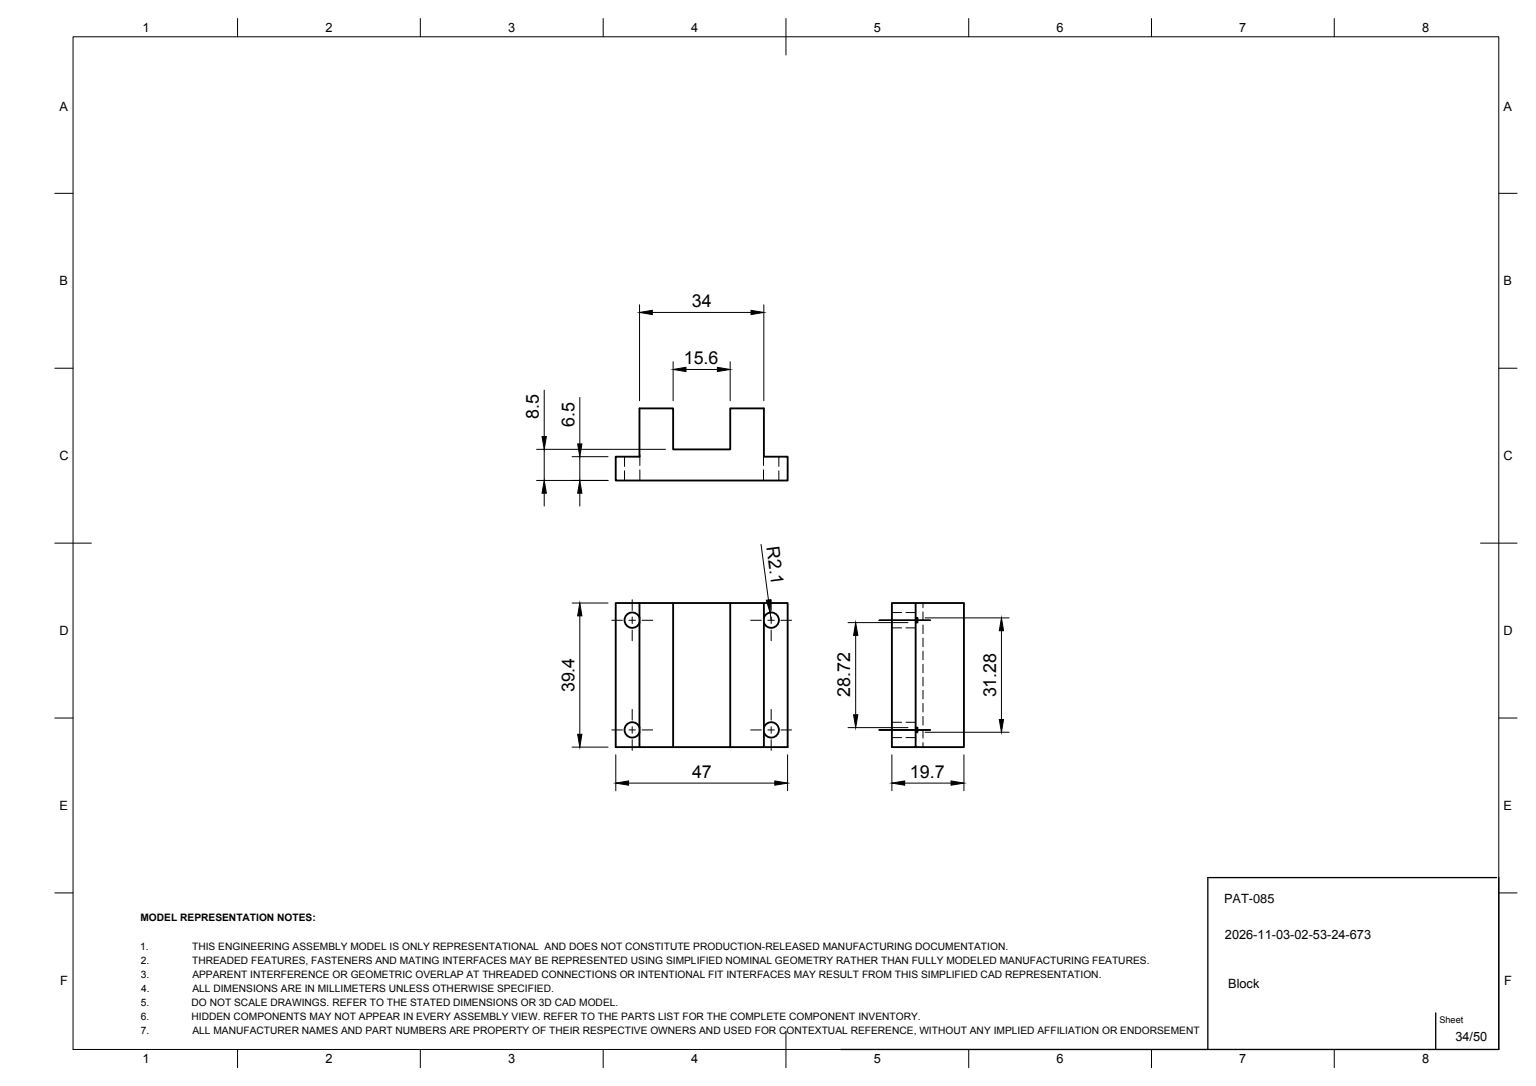
ISO-10303-21;
HEADER;
/* Generated by software containing ST-Developer
 * from STEP Tools, Inc. (www.steptools.com) 
 */

FILE_DESCRIPTION(
/* description */ ('Rack and pinion manual slide'),
/* implementation_level */ '2;1');

FILE_NAME(
/* name */ 'Block.step',
/* time_stamp */ '2026-10-28T03:22:49-07:00',
/* author */ (''),
/* organization */ (''),
/* preprocessor_version */ 'ST-DEVELOPER v20.2',
/* originating_system */ 'Autodesk Translation Framework v15.17.0.0',
/* authorisation */ '');

FILE_SCHEMA (('AUTOMOTIVE_DESIGN { 1 0 10303 214 3 1 1 }'));
ENDSEC;

DATA;
#10=MECHANICAL_DESIGN_GEOMETRIC_PRESENTATION_REPRESENTATION('',(#766),#34851);
#667=SHAPE_REPRESENTATION_RELATIONSHIP('SRR','None',#35105,#713);
#713=ADVANCED_BREP_SHAPE_REPRESENTATION('',(#817),#34830);
#766=STYLED_ITEM('',(#35390),#817);
#817=MANIFOLD_SOLID_BREP('Body1',#13788);
#1005=FACE_BOUND('',#2939,.T.);
#1006=FACE_BOUND('',#2940,.T.);
#1007=FACE_BOUND('',#2941,.T.);
#1008=FACE_BOUND('',#2942,.T.);
#1385=PLANE('',#15111);
#1386=PLANE('',#15117);
#1387=PLANE('',#15123);
#1388=PLANE('',#15129);
#1389=PLANE('',#15135);
#1390=PLANE('',#15136);
#1391=PLANE('',#15137);
#1392=PLANE('',#15138);
#1393=PLANE('',#15139);
#1394=PLANE('',#15140);
#1395=PLANE('',#15141);
#1396=PLANE('',#15142);
#1397=PLANE('',#15143);
#1398=PLANE('',#15144);
#1399=PLANE('',#15145);
#1400=PLANE('',#15146);
#1401=PLANE('',#15147);
#1402=PLANE('',#15148);
#2014=FACE_OUTER_BOUND('',#2925,.T.);
#2015=FACE_OUTER_BOUND('',#2926,.T.);
#2016=FACE_OUTER_BOUND('',#2927,.T.);
#2017=FACE_OUTER_BOUND('',#2928,.T.);
#2018=FACE_OUTER_BOUND('',#2929,.T.);
#2019=FACE_OUTER_BOUND('',#2930,.T.);
#2020=FACE_OUTER_BOUND('',#2931,.T.);
#2021=FACE_OUTER_BOUND('',#2932,.T.);
#2022=FACE_OUTER_BOUND('',#2933,.T.);
#2023=FACE_OUTER_BOUND('',#2934,.T.);
#2024=FACE_OUTER_BOUND('',#2935,.T.);
#2025=FACE_OUTER_BOUND('',#2936,.T.);
#2026=FACE_OUTER_BOUND('',#2937,.T.);
#2027=FACE_OUTER_BOUND('',#2938,.T.);
#2028=FACE_OUTER_BOUND('',#2943,.T.);
#2029=FACE_OUTER_BOUND('',#2944,.T.);
#2030=FACE_OUTER_BOUND('',#2945,.T.);
#2031=FACE_OUTER_BOUND('',#2946,.T.);
#2032=FACE_OUTER_BOUND('',#2947,.T.);
#2033=FACE_OUTER_BOUND('',#2948,.T.);
#2034=FACE_OUTER_BOUND('',#2949,.T.);
#2035=FACE_OUTER_BOUND('',#2950,.T.);
#2925=EDGE_LOOP('',(#11612,#11613));
#2926=EDGE_LOOP('',(#11614,#11615,#11616,#11617,#11618,#11619,#11620,#11621));
#2927=EDGE_LOOP('',(#11622,#11623));
#2928=EDGE_LOOP('',(#11624,#11625,#11626,#11627,#11628,#11629,#11630,#11631));
#2929=EDGE_LOOP('',(#11632,#11633));
#2930=EDGE_LOOP('',(#11634,#11635,#11636,#11637,#11638,#11639,#11640,#11641));
#2931=EDGE_LOOP('',(#11642,#11643));
#2932=EDGE_LOOP('',(#11644,#11645,#11646,#11647,#11648,#11649,#11650,#11651));
#2933=EDGE_LOOP('',(#11652,#11653,#11654,#11655,#11656,#11657,#11658,#11659,
#11660,#11661,#11662,#11663));
#2934=EDGE_LOOP('',(#11664,#11665,#11666,#11667,#11668,#11669,#11670,#11671,
#11672,#11673,#11674,#11675));
#2935=EDGE_LOOP('',(#11676,#11677,#11678,#11679,#11680,#11681,#11682,#11683,
#11684,#11685,#11686,#11687));
#2936=EDGE_LOOP('',(#11688,#11689,#11690,#11691,#11692,#11693,#11694,#11695,
#11696,#11697));
#2937=EDGE_LOOP('',(#11698,#11699,#11700,#11701));
#2938=EDGE_LOOP('',(#11702,#11703,#11704,#11705));
#2939=EDGE_LOOP('',(#11706));
#2940=EDGE_LOOP('',(#11707));
#2941=EDGE_LOOP('',(#11708));
#2942=EDGE_LOOP('',(#11709));
#2943=EDGE_LOOP('',(#11710,#11711,#11712,#11713));
#2944=EDGE_LOOP('',(#11714,#11715,#11716,#11717,#11718,#11719,#11720,#11721,
#11722,#11723));
#2945=EDGE_LOOP('',(#11724,#11725,#11726,#11727));
#2946=EDGE_LOOP('',(#11728,#11729,#11730,#11731));
#2947=EDGE_LOOP('',(#11732,#11733,#11734,#11735));
#2948=EDGE_LOOP('',(#11736,#11737,#11738,#11739));
#2949=EDGE_LOOP('',(#11740,#11741,#11742,#11743));
#2950=EDGE_LOOP('',(#11744,#11745,#11746,#11747,#11748,#11749,#11750,#11751,
#11752,#11753,#11754,#11755));
#4122=LINE('',#22258,#5413);
#4123=LINE('',#22262,#5414);
#4124=LINE('',#22266,#5415);
#4125=LINE('',#22270,#5416);
#4126=LINE('',#22274,#5417);
#4127=LINE('',#22278,#5418);
#4128=LINE('',#22282,#5419);
#4129=LINE('',#22286,#5420);
#4130=LINE('',#22290,#5421);
#4131=LINE('',#22294,#5422);
#4132=LINE('',#22298,#5423);
#4133=LINE('',#22302,#5424);
#4134=LINE('',#22306,#5425);
#4135=LINE('',#22310,#5426);
#4136=LINE('',#22314,#5427);
#4137=LINE('',#22318,#5428);
#4138=LINE('',#22320,#5429);
#4139=LINE('',#22322,#5430);
#4140=LINE('',#22324,#5431);
#4141=LINE('',#22326,#5432);
#4142=LINE('',#22328,#5433);
#4143=LINE('',#22329,#5434);
#4144=LINE('',#22331,#5435);
#4145=LINE('',#22333,#5436);
#4146=LINE('',#22335,#5437);
#4147=LINE('',#22337,#5438);
#4148=LINE('',#22339,#5439);
#4149=LINE('',#22340,#5440);
#4150=LINE('',#22343,#5441);
#4151=LINE('',#22345,#5442);
#4152=LINE('',#22347,#5443);
#4153=LINE('',#22349,#5444);
#4154=LINE('',#22350,#5445);
#4155=LINE('',#22352,#5446);
#4156=LINE('',#22354,#5447);
#4157=LINE('',#22356,#5448);
#4158=LINE('',#22358,#5449);
#4159=LINE('',#22359,#5450);
#4160=LINE('',#22362,#5451);
#4161=LINE('',#22363,#5452);
#4162=LINE('',#22366,#5453);
#4163=LINE('',#22367,#5454);
#4164=LINE('',#22370,#5455);
#4165=LINE('',#22371,#5456);
#4166=LINE('',#22374,#5457);
#4167=LINE('',#22375,#5458);
#4168=LINE('',#22377,#5459);
#4169=LINE('',#22380,#5460);
#4170=LINE('',#22381,#5461);
#4171=LINE('',#22384,#5462);
#4172=LINE('',#22385,#5463);
#4173=LINE('',#22388,#5464);
#4174=LINE('',#22389,#5465);
#4175=LINE('',#22392,#5466);
#4176=LINE('',#22393,#5467);
#4177=LINE('',#22395,#5468);
#5413=VECTOR('',#18088,1.);
#5414=VECTOR('',#18093,1.);
#5415=VECTOR('',#18096,0.21);
#5416=VECTOR('',#18101,1.);
#5417=VECTOR('',#18104,1.);
#5418=VECTOR('',#18109,1.);
#5419=VECTOR('',#18112,0.21);
#5420=VECTOR('',#18117,1.);
#5421=VECTOR('',#18120,1.);
#5422=VECTOR('',#18125,1.);
#5423=VECTOR('',#18128,0.21);
#5424=VECTOR('',#18133,1.);
#5425=VECTOR('',#18136,1.);
#5426=VECTOR('',#18141,1.);
#5427=VECTOR('',#18144,0.21);
#5428=VECTOR('',#18149,1.);
#5429=VECTOR('',#18152,1.);
#5430=VECTOR('',#18153,1.);
#5431=VECTOR('',#18154,1.);
#5432=VECTOR('',#18155,1.);
#5433=VECTOR('',#18156,1.);
#5434=VECTOR('',#18157,1.);
#5435=VECTOR('',#18160,1.);
#5436=VECTOR('',#18161,1.);
#5437=VECTOR('',#18162,1.);
#5438=VECTOR('',#18163,1.);
#5439=VECTOR('',#18164,1.);
#5440=VECTOR('',#18165,1.);
#5441=VECTOR('',#18168,1.);
#5442=VECTOR('',#18169,1.);
#5443=VECTOR('',#18170,1.);
#5444=VECTOR('',#18171,1.);
#5445=VECTOR('',#18172,1.);
#5446=VECTOR('',#18173,1.);
#5447=VECTOR('',#18174,1.);
#5448=VECTOR('',#18175,1.);
#5449=VECTOR('',#18176,1.);
#5450=VECTOR('',#18177,1.);
#5451=VECTOR('',#18180,1.);
#5452=VECTOR('',#18181,1.);
#5453=VECTOR('',#18184,1.);
#5454=VECTOR('',#18185,1.);
#5455=VECTOR('',#18188,1.);
#5456=VECTOR('',#18189,1.);
#5457=VECTOR('',#18192,1.);
#5458=VECTOR('',#18193,1.);
#5459=VECTOR('',#18196,1.);
#5460=VECTOR('',#18199,1.);
#5461=VECTOR('',#18200,1.);
#5462=VECTOR('',#18203,1.);
#5463=VECTOR('',#18204,1.);
#5464=VECTOR('',#18207,1.);
#5465=VECTOR('',#18208,1.);
#5466=VECTOR('',#18211,1.);
#5467=VECTOR('',#18212,1.);
#5468=VECTOR('',#18215,1.);
#6081=CIRCLE('',#15112,0.21);
#6082=CIRCLE('',#15114,0.21);
#6083=CIRCLE('',#15115,0.21);
#6084=CIRCLE('',#15116,0.21);
#6085=CIRCLE('',#15118,0.21);
#6086=CIRCLE('',#15120,0.21);
#6087=CIRCLE('',#15121,0.21);
#6088=CIRCLE('',#15122,0.21);
#6089=CIRCLE('',#15124,0.21);
#6090=CIRCLE('',#15126,0.21);
#6091=CIRCLE('',#15127,0.21);
#6092=CIRCLE('',#15128,0.21);
#6093=CIRCLE('',#15130,0.21);
#6094=CIRCLE('',#15132,0.21);
#6095=CIRCLE('',#15133,0.21);
#6096=CIRCLE('',#15134,0.21);
#7022=VERTEX_POINT('',#22256);
#7023=VERTEX_POINT('',#22257);
#7024=VERTEX_POINT('',#22261);
#7025=VERTEX_POINT('',#22263);
#7026=VERTEX_POINT('',#22265);
#7027=VERTEX_POINT('',#22268);
#7028=VERTEX_POINT('',#22272);
#7029=VERTEX_POINT('',#22273);
#7030=VERTEX_POINT('',#22277);
#7031=VERTEX_POINT('',#22279);
#7032=VERTEX_POINT('',#22281);
#7033=VERTEX_POINT('',#22284);
#7034=VERTEX_POINT('',#22288);
#7035=VERTEX_POINT('',#22289);
#7036=VERTEX_POINT('',#22293);
#7037=VERTEX_POINT('',#22295);
#7038=VERTEX_POINT('',#22297);
#7039=VERTEX_POINT('',#22300);
#7040=VERTEX_POINT('',#22304);
#7041=VERTEX_POINT('',#22305);
#7042=VERTEX_POINT('',#22309);
#7043=VERTEX_POINT('',#22311);
#7044=VERTEX_POINT('',#22313);
#7045=VERTEX_POINT('',#22316);
#7046=VERTEX_POINT('',#22321);
#7047=VERTEX_POINT('',#22323);
#7048=VERTEX_POINT('',#22325);
#7049=VERTEX_POINT('',#22327);
#7050=VERTEX_POINT('',#22332);
#7051=VERTEX_POINT('',#22334);
#7052=VERTEX_POINT('',#22336);
#7053=VERTEX_POINT('',#22338);
#7054=VERTEX_POINT('',#22342);
#7055=VERTEX_POINT('',#22344);
#7056=VERTEX_POINT('',#22346);
#7057=VERTEX_POINT('',#22348);
#7058=VERTEX_POINT('',#22351);
#7059=VERTEX_POINT('',#22353);
#7060=VERTEX_POINT('',#22355);
#7061=VERTEX_POINT('',#22357);
#7062=VERTEX_POINT('',#22361);
#7063=VERTEX_POINT('',#22365);
#7064=VERTEX_POINT('',#22369);
#7065=VERTEX_POINT('',#22373);
#7066=VERTEX_POINT('',#22379);
#7067=VERTEX_POINT('',#22383);
#7068=VERTEX_POINT('',#22387);
#7069=VERTEX_POINT('',#22391);
#8618=EDGE_CURVE('',#7022,#7023,#4122,.T.);
#8619=EDGE_CURVE('',#7022,#7023,#6081,.T.);
#8620=EDGE_CURVE('',#7024,#7022,#4123,.T.);
#8621=EDGE_CURVE('',#7025,#7024,#6082,.T.);
#8622=EDGE_CURVE('',#7025,#7026,#4124,.T.);
#8623=EDGE_CURVE('',#7026,#7026,#6083,.T.);
#8624=EDGE_CURVE('',#7027,#7025,#6084,.T.);
#8625=EDGE_CURVE('',#7023,#7027,#4125,.T.);
#8626=EDGE_CURVE('',#7028,#7029,#4126,.T.);
#8627=EDGE_CURVE('',#7028,#7029,#6085,.T.);
#8628=EDGE_CURVE('',#7030,#7028,#4127,.T.);
#8629=EDGE_CURVE('',#7031,#7030,#6086,.T.);
#8630=EDGE_CURVE('',#7031,#7032,#4128,.T.);
#8631=EDGE_CURVE('',#7032,#7032,#6087,.T.);
#8632=EDGE_CURVE('',#7033,#7031,#6088,.T.);
#8633=EDGE_CURVE('',#7029,#7033,#4129,.T.);
#8634=EDGE_CURVE('',#7034,#7035,#4130,.T.);
#8635=EDGE_CURVE('',#7034,#7035,#6089,.T.);
#8636=EDGE_CURVE('',#7036,#7034,#4131,.T.);
#8637=EDGE_CURVE('',#7037,#7036,#6090,.T.);
#8638=EDGE_CURVE('',#7037,#7038,#4132,.T.);
#8639=EDGE_CURVE('',#7038,#7038,#6091,.T.);
#8640=EDGE_CURVE('',#7039,#7037,#6092,.T.);
#8641=EDGE_CURVE('',#7035,#7039,#4133,.T.);
#8642=EDGE_CURVE('',#7040,#7041,#4134,.T.);
#8643=EDGE_CURVE('',#7040,#7041,#6093,.T.);
#8644=EDGE_CURVE('',#7042,#7040,#4135,.T.);
#8645=EDGE_CURVE('',#7043,#7042,#6094,.T.);
#8646=EDGE_CURVE('',#7043,#7044,#4136,.T.);
#8647=EDGE_CURVE('',#7044,#7044,#6095,.T.);
#8648=EDGE_CURVE('',#7045,#7043,#6096,.T.);
#8649=EDGE_CURVE('',#7041,#7045,#4137,.T.);
#8650=EDGE_CURVE('',#7027,#7036,#4138,.T.);
#8651=EDGE_CURVE('',#7039,#7046,#4139,.T.);
#8652=EDGE_CURVE('',#7047,#7046,#4140,.T.);
#8653=EDGE_CURVE('',#7047,#7048,#4141,.T.);
#8654=EDGE_CURVE('',#7049,#7048,#4142,.T.);
#8655=EDGE_CURVE('',#7049,#7024,#4143,.T.);
#8656=EDGE_CURVE('',#7033,#7042,#4144,.T.);
#8657=EDGE_CURVE('',#7045,#7050,#4145,.T.);
#8658=EDGE_CURVE('',#7051,#7050,#4146,.T.);
#8659=EDGE_CURVE('',#7052,#7051,#4147,.T.);
#8660=EDGE_CURVE('',#7053,#7052,#4148,.T.);
#8661=EDGE_CURVE('',#7053,#7030,#4149,.T.);
#8662=EDGE_CURVE('',#7046,#7054,#4150,.T.);
#8663=EDGE_CURVE('',#7054,#7055,#4151,.T.);
#8664=EDGE_CURVE('',#7055,#7056,#4152,.T.);
#8665=EDGE_CURVE('',#7056,#7057,#4153,.T.);
#8666=EDGE_CURVE('',#7057,#7053,#4154,.T.);
#8667=EDGE_CURVE('',#7052,#7058,#4155,.T.);
#8668=EDGE_CURVE('',#7058,#7059,#4156,.T.);
#8669=EDGE_CURVE('',#7059,#7060,#4157,.T.);
#8670=EDGE_CURVE('',#7060,#7061,#4158,.T.);
#8671=EDGE_CURVE('',#7061,#7047,#4159,.T.);
#8672=EDGE_CURVE('',#7062,#7049,#4160,.T.);
#8673=EDGE_CURVE('',#7054,#7062,#4161,.T.);
#8674=EDGE_CURVE('',#7063,#7062,#4162,.T.);
#8675=EDGE_CURVE('',#7055,#7063,#4163,.T.);
#8676=EDGE_CURVE('',#7064,#7063,#4164,.T.);
#8677=EDGE_CURVE('',#7056,#7064,#4165,.T.);
#8678=EDGE_CURVE('',#7065,#7064,#4166,.T.);
#8679=EDGE_CURVE('',#7057,#7065,#4167,.T.);
#8680=EDGE_CURVE('',#7050,#7065,#4168,.T.);
#8681=EDGE_CURVE('',#7066,#7051,#4169,.T.);
#8682=EDGE_CURVE('',#7058,#7066,#4170,.T.);
#8683=EDGE_CURVE('',#7067,#7066,#4171,.T.);
#8684=EDGE_CURVE('',#7059,#7067,#4172,.T.);
#8685=EDGE_CURVE('',#7068,#7067,#4173,.T.);
#8686=EDGE_CURVE('',#7060,#7068,#4174,.T.);
#8687=EDGE_CURVE('',#7069,#7068,#4175,.T.);
#8688=EDGE_CURVE('',#7061,#7069,#4176,.T.);
#8689=EDGE_CURVE('',#7048,#7069,#4177,.T.);
#11612=ORIENTED_EDGE('',*,*,#8618,.F.);
#11613=ORIENTED_EDGE('',*,*,#8619,.T.);
#11614=ORIENTED_EDGE('',*,*,#8620,.F.);
#11615=ORIENTED_EDGE('',*,*,#8621,.F.);
#11616=ORIENTED_EDGE('',*,*,#8622,.T.);
#11617=ORIENTED_EDGE('',*,*,#8623,.F.);
#11618=ORIENTED_EDGE('',*,*,#8622,.F.);
#11619=ORIENTED_EDGE('',*,*,#8624,.F.);
#11620=ORIENTED_EDGE('',*,*,#8625,.F.);
#11621=ORIENTED_EDGE('',*,*,#8619,.F.);
#11622=ORIENTED_EDGE('',*,*,#8626,.F.);
#11623=ORIENTED_EDGE('',*,*,#8627,.T.);
#11624=ORIENTED_EDGE('',*,*,#8628,.F.);
#11625=ORIENTED_EDGE('',*,*,#8629,.F.);
#11626=ORIENTED_EDGE('',*,*,#8630,.T.);
#11627=ORIENTED_EDGE('',*,*,#8631,.F.);
#11628=ORIENTED_EDGE('',*,*,#8630,.F.);
#11629=ORIENTED_EDGE('',*,*,#8632,.F.);
#11630=ORIENTED_EDGE('',*,*,#8633,.F.);
#11631=ORIENTED_EDGE('',*,*,#8627,.F.);
#11632=ORIENTED_EDGE('',*,*,#8634,.F.);
#11633=ORIENTED_EDGE('',*,*,#8635,.T.);
#11634=ORIENTED_EDGE('',*,*,#8636,.F.);
#11635=ORIENTED_EDGE('',*,*,#8637,.F.);
#11636=ORIENTED_EDGE('',*,*,#8638,.T.);
#11637=ORIENTED_EDGE('',*,*,#8639,.F.);
#11638=ORIENTED_EDGE('',*,*,#8638,.F.);
#11639=ORIENTED_EDGE('',*,*,#8640,.F.);
#11640=ORIENTED_EDGE('',*,*,#8641,.F.);
#11641=ORIENTED_EDGE('',*,*,#8635,.F.);
#11642=ORIENTED_EDGE('',*,*,#8642,.F.);
#11643=ORIENTED_EDGE('',*,*,#8643,.T.);
#11644=ORIENTED_EDGE('',*,*,#8644,.F.);
#11645=ORIENTED_EDGE('',*,*,#8645,.F.);
#11646=ORIENTED_EDGE('',*,*,#8646,.T.);
#11647=ORIENTED_EDGE('',*,*,#8647,.F.);
#11648=ORIENTED_EDGE('',*,*,#8646,.F.);
#11649=ORIENTED_EDGE('',*,*,#8648,.F.);
#11650=ORIENTED_EDGE('',*,*,#8649,.F.);
#11651=ORIENTED_EDGE('',*,*,#8643,.F.);
#11652=ORIENTED_EDGE('',*,*,#8620,.T.);
#11653=ORIENTED_EDGE('',*,*,#8618,.T.);
#11654=ORIENTED_EDGE('',*,*,#8625,.T.);
#11655=ORIENTED_EDGE('',*,*,#8650,.T.);
#11656=ORIENTED_EDGE('',*,*,#8636,.T.);
#11657=ORIENTED_EDGE('',*,*,#8634,.T.);
#11658=ORIENTED_EDGE('',*,*,#8641,.T.);
#11659=ORIENTED_EDGE('',*,*,#8651,.T.);
#11660=ORIENTED_EDGE('',*,*,#8652,.F.);
#11661=ORIENTED_EDGE('',*,*,#8653,.T.);
#11662=ORIENTED_EDGE('',*,*,#8654,.F.);
#11663=ORIENTED_EDGE('',*,*,#8655,.T.);
#11664=ORIENTED_EDGE('',*,*,#8628,.T.);
#11665=ORIENTED_EDGE('',*,*,#8626,.T.);
#11666=ORIENTED_EDGE('',*,*,#8633,.T.);
#11667=ORIENTED_EDGE('',*,*,#8656,.T.);
#11668=ORIENTED_EDGE('',*,*,#8644,.T.);
#11669=ORIENTED_EDGE('',*,*,#8642,.T.);
#11670=ORIENTED_EDGE('',*,*,#8649,.T.);
#11671=ORIENTED_EDGE('',*,*,#8657,.T.);
#11672=ORIENTED_EDGE('',*,*,#8658,.F.);
#11673=ORIENTED_EDGE('',*,*,#8659,.F.);
#11674=ORIENTED_EDGE('',*,*,#8660,.F.);
#11675=ORIENTED_EDGE('',*,*,#8661,.T.);
#11676=ORIENTED_EDGE('',*,*,#8652,.T.);
#11677=ORIENTED_EDGE('',*,*,#8662,.T.);
#11678=ORIENTED_EDGE('',*,*,#8663,.T.);
#11679=ORIENTED_EDGE('',*,*,#8664,.T.);
#11680=ORIENTED_EDGE('',*,*,#8665,.T.);
#11681=ORIENTED_EDGE('',*,*,#8666,.T.);
#11682=ORIENTED_EDGE('',*,*,#8660,.T.);
#11683=ORIENTED_EDGE('',*,*,#8667,.T.);
#11684=ORIENTED_EDGE('',*,*,#8668,.T.);
#11685=ORIENTED_EDGE('',*,*,#8669,.T.);
#11686=ORIENTED_EDGE('',*,*,#8670,.T.);
#11687=ORIENTED_EDGE('',*,*,#8671,.T.);
#11688=ORIENTED_EDGE('',*,*,#8624,.T.);
#11689=ORIENTED_EDGE('',*,*,#8621,.T.);
#11690=ORIENTED_EDGE('',*,*,#8655,.F.);
#11691=ORIENTED_EDGE('',*,*,#8672,.F.);
#11692=ORIENTED_EDGE('',*,*,#8673,.F.);
#11693=ORIENTED_EDGE('',*,*,#8662,.F.);
#11694=ORIENTED_EDGE('',*,*,#8651,.F.);
#11695=ORIENTED_EDGE('',*,*,#8640,.T.);
#11696=ORIENTED_EDGE('',*,*,#8637,.T.);
#11697=ORIENTED_EDGE('',*,*,#8650,.F.);
#11698=ORIENTED_EDGE('',*,*,#8673,.T.);
#11699=ORIENTED_EDGE('',*,*,#8674,.F.);
#11700=ORIENTED_EDGE('',*,*,#8675,.F.);
#11701=ORIENTED_EDGE('',*,*,#8663,.F.);
#11702=ORIENTED_EDGE('',*,*,#8675,.T.);
#11703=ORIENTED_EDGE('',*,*,#8676,.F.);
#11704=ORIENTED_EDGE('',*,*,#8677,.F.);
#11705=ORIENTED_EDGE('',*,*,#8664,.F.);
#11706=ORIENTED_EDGE('',*,*,#8623,.T.);
#11707=ORIENTED_EDGE('',*,*,#8631,.T.);
#11708=ORIENTED_EDGE('',*,*,#8639,.T.);
#11709=ORIENTED_EDGE('',*,*,#8647,.T.);
#11710=ORIENTED_EDGE('',*,*,#8677,.T.);
#11711=ORIENTED_EDGE('',*,*,#8678,.F.);
#11712=ORIENTED_EDGE('',*,*,#8679,.F.);
#11713=ORIENTED_EDGE('',*,*,#8665,.F.);
#11714=ORIENTED_EDGE('',*,*,#8632,.T.);
#11715=ORIENTED_EDGE('',*,*,#8629,.T.);
#11716=ORIENTED_EDGE('',*,*,#8661,.F.);
#11717=ORIENTED_EDGE('',*,*,#8666,.F.);
#11718=ORIENTED_EDGE('',*,*,#8679,.T.);
#11719=ORIENTED_EDGE('',*,*,#8680,.F.);
#11720=ORIENTED_EDGE('',*,*,#8657,.F.);
#11721=ORIENTED_EDGE('',*,*,#8648,.T.);
#11722=ORIENTED_EDGE('',*,*,#8645,.T.);
#11723=ORIENTED_EDGE('',*,*,#8656,.F.);
#11724=ORIENTED_EDGE('',*,*,#8659,.T.);
#11725=ORIENTED_EDGE('',*,*,#8681,.F.);
#11726=ORIENTED_EDGE('',*,*,#8682,.F.);
#11727=ORIENTED_EDGE('',*,*,#8667,.F.);
#11728=ORIENTED_EDGE('',*,*,#8682,.T.);
#11729=ORIENTED_EDGE('',*,*,#8683,.F.);
#11730=ORIENTED_EDGE('',*,*,#8684,.F.);
#11731=ORIENTED_EDGE('',*,*,#8668,.F.);
#11732=ORIENTED_EDGE('',*,*,#8684,.T.);
#11733=ORIENTED_EDGE('',*,*,#8685,.F.);
#11734=ORIENTED_EDGE('',*,*,#8686,.F.);
#11735=ORIENTED_EDGE('',*,*,#8669,.F.);
#11736=ORIENTED_EDGE('',*,*,#8686,.T.);
#11737=ORIENTED_EDGE('',*,*,#8687,.F.);
#11738=ORIENTED_EDGE('',*,*,#8688,.F.);
#11739=ORIENTED_EDGE('',*,*,#8670,.F.);
#11740=ORIENTED_EDGE('',*,*,#8688,.T.);
#11741=ORIENTED_EDGE('',*,*,#8689,.F.);
#11742=ORIENTED_EDGE('',*,*,#8653,.F.);
#11743=ORIENTED_EDGE('',*,*,#8671,.F.);
#11744=ORIENTED_EDGE('',*,*,#8654,.T.);
#11745=ORIENTED_EDGE('',*,*,#8689,.T.);
#11746=ORIENTED_EDGE('',*,*,#8687,.T.);
#11747=ORIENTED_EDGE('',*,*,#8685,.T.);
#11748=ORIENTED_EDGE('',*,*,#8683,.T.);
#11749=ORIENTED_EDGE('',*,*,#8681,.T.);
#11750=ORIENTED_EDGE('',*,*,#8658,.T.);
#11751=ORIENTED_EDGE('',*,*,#8680,.T.);
#11752=ORIENTED_EDGE('',*,*,#8678,.T.);
#11753=ORIENTED_EDGE('',*,*,#8676,.T.);
#11754=ORIENTED_EDGE('',*,*,#8674,.T.);
#11755=ORIENTED_EDGE('',*,*,#8672,.T.);
#12954=CYLINDRICAL_SURFACE('',#15113,0.21);
#12955=CYLINDRICAL_SURFACE('',#15119,0.21);
#12956=CYLINDRICAL_SURFACE('',#15125,0.21);
#12957=CYLINDRICAL_SURFACE('',#15131,0.21);
#13492=ADVANCED_FACE('',(#2014),#1385,.T.);
#13493=ADVANCED_FACE('',(#2015),#12954,.F.);
#13494=ADVANCED_FACE('',(#2016),#1386,.T.);
#13495=ADVANCED_FACE('',(#2017),#12955,.F.);
#13496=ADVANCED_FACE('',(#2018),#1387,.T.);
#13497=ADVANCED_FACE('',(#2019),#12956,.F.);
#13498=ADVANCED_FACE('',(#2020),#1388,.T.);
#13499=ADVANCED_FACE('',(#2021),#12957,.F.);
#13500=ADVANCED_FACE('',(#2022),#1389,.T.);
#13501=ADVANCED_FACE('',(#2023),#1390,.T.);
#13502=ADVANCED_FACE('',(#2024),#1391,.T.);
#13503=ADVANCED_FACE('',(#2025),#1392,.T.);
#13504=ADVANCED_FACE('',(#2026),#1393,.T.);
#13505=ADVANCED_FACE('',(#2027,#1005,#1006,#1007,#1008),#1394,.T.);
#13506=ADVANCED_FACE('',(#2028),#1395,.T.);
#13507=ADVANCED_FACE('',(#2029),#1396,.T.);
#13508=ADVANCED_FACE('',(#2030),#1397,.T.);
#13509=ADVANCED_FACE('',(#2031),#1398,.T.);
#13510=ADVANCED_FACE('',(#2032),#1399,.T.);
#13511=ADVANCED_FACE('',(#2033),#1400,.T.);
#13512=ADVANCED_FACE('',(#2034),#1401,.T.);
#13513=ADVANCED_FACE('',(#2035),#1402,.T.);
#13788=CLOSED_SHELL('',(#13492,#13493,#13494,#13495,#13496,#13497,#13498,
#13499,#13500,#13501,#13502,#13503,#13504,#13505,#13506,#13507,#13508,#13509,
#13510,#13511,#13512,#13513));
#15110=AXIS2_PLACEMENT_3D('',#22254,#18084,#18085);
#15111=AXIS2_PLACEMENT_3D('',#22255,#18086,#18087);
#15112=AXIS2_PLACEMENT_3D('',#22259,#18089,#18090);
#15113=AXIS2_PLACEMENT_3D('',#22260,#18091,#18092);
#15114=AXIS2_PLACEMENT_3D('',#22264,#18094,#18095);
#15115=AXIS2_PLACEMENT_3D('',#22267,#18097,#18098);
#15116=AXIS2_PLACEMENT_3D('',#22269,#18099,#18100);
#15117=AXIS2_PLACEMENT_3D('',#22271,#18102,#18103);
#15118=AXIS2_PLACEMENT_3D('',#22275,#18105,#18106);
#15119=AXIS2_PLACEMENT_3D('',#22276,#18107,#18108);
#15120=AXIS2_PLACEMENT_3D('',#22280,#18110,#18111);
#15121=AXIS2_PLACEMENT_3D('',#22283,#18113,#18114);
#15122=AXIS2_PLACEMENT_3D('',#22285,#18115,#18116);
#15123=AXIS2_PLACEMENT_3D('',#22287,#18118,#18119);
#15124=AXIS2_PLACEMENT_3D('',#22291,#18121,#18122);
#15125=AXIS2_PLACEMENT_3D('',#22292,#18123,#18124);
#15126=AXIS2_PLACEMENT_3D('',#22296,#18126,#18127);
#15127=AXIS2_PLACEMENT_3D('',#22299,#18129,#18130);
#15128=AXIS2_PLACEMENT_3D('',#22301,#18131,#18132);
#15129=AXIS2_PLACEMENT_3D('',#22303,#18134,#18135);
#15130=AXIS2_PLACEMENT_3D('',#22307,#18137,#18138);
#15131=AXIS2_PLACEMENT_3D('',#22308,#18139,#18140);
#15132=AXIS2_PLACEMENT_3D('',#22312,#18142,#18143);
#15133=AXIS2_PLACEMENT_3D('',#22315,#18145,#18146);
#15134=AXIS2_PLACEMENT_3D('',#22317,#18147,#18148);
#15135=AXIS2_PLACEMENT_3D('',#22319,#18150,#18151);
#15136=AXIS2_PLACEMENT_3D('',#22330,#18158,#18159);
#15137=AXIS2_PLACEMENT_3D('',#22341,#18166,#18167);
#15138=AXIS2_PLACEMENT_3D('',#22360,#18178,#18179);
#15139=AXIS2_PLACEMENT_3D('',#22364,#18182,#18183);
#15140=AXIS2_PLACEMENT_3D('',#22368,#18186,#18187);
#15141=AXIS2_PLACEMENT_3D('',#22372,#18190,#18191);
#15142=AXIS2_PLACEMENT_3D('',#22376,#18194,#18195);
#15143=AXIS2_PLACEMENT_3D('',#22378,#18197,#18198);
#15144=AXIS2_PLACEMENT_3D('',#22382,#18201,#18202);
#15145=AXIS2_PLACEMENT_3D('',#22386,#18205,#18206);
#15146=AXIS2_PLACEMENT_3D('',#22390,#18209,#18210);
#15147=AXIS2_PLACEMENT_3D('',#22394,#18213,#18214);
#15148=AXIS2_PLACEMENT_3D('',#22396,#18216,#18217);
#18084=DIRECTION('axis',(0.,0.,1.));
#18085=DIRECTION('refdir',(1.,0.,0.));
#18086=DIRECTION('center_axis',(0.,0.,1.));
#18087=DIRECTION('ref_axis',(1.,0.,0.));
#18088=DIRECTION('',(-1.,0.,0.));
#18089=DIRECTION('center_axis',(0.,0.,1.));
#18090=DIRECTION('ref_axis',(1.,0.,0.));
#18091=DIRECTION('center_axis',(0.,0.,1.));
#18092=DIRECTION('ref_axis',(1.,0.,0.));
#18093=DIRECTION('',(0.,0.,-1.));
#18094=DIRECTION('center_axis',(0.,0.,1.));
#18095=DIRECTION('ref_axis',(1.,0.,0.));
#18096=DIRECTION('',(0.,0.,1.));
#18097=DIRECTION('center_axis',(0.,0.,-1.));
#18098=DIRECTION('ref_axis',(1.,0.,0.));
#18099=DIRECTION('center_axis',(0.,0.,1.));
#18100=DIRECTION('ref_axis',(1.,0.,0.));
#18101=DIRECTION('',(0.,0.,1.));
#18102=DIRECTION('center_axis',(0.,0.,1.));
#18103=DIRECTION('ref_axis',(1.,0.,0.));
#18104=DIRECTION('',(1.,0.,0.));
#18105=DIRECTION('center_axis',(0.,0.,1.));
#18106=DIRECTION('ref_axis',(1.,0.,0.));
#18107=DIRECTION('center_axis',(0.,0.,1.));
#18108=DIRECTION('ref_axis',(1.,0.,0.));
#18109=DIRECTION('',(0.,0.,-1.));
#18110=DIRECTION('center_axis',(0.,0.,1.));
#18111=DIRECTION('ref_axis',(1.,0.,0.));
#18112=DIRECTION('',(0.,0.,1.));
#18113=DIRECTION('center_axis',(0.,0.,-1.));
#18114=DIRECTION('ref_axis',(1.,0.,0.));
#18115=DIRECTION('center_axis',(0.,0.,1.));
#18116=DIRECTION('ref_axis',(1.,0.,0.));
#18117=DIRECTION('',(0.,0.,1.));
#18118=DIRECTION('center_axis',(0.,0.,1.));
#18119=DIRECTION('ref_axis',(1.,0.,0.));
#18120=DIRECTION('',(-1.,0.,0.));
#18121=DIRECTION('center_axis',(0.,0.,1.));
#18122=DIRECTION('ref_axis',(1.,0.,0.));
#18123=DIRECTION('center_axis',(0.,0.,1.));
#18124=DIRECTION('ref_axis',(1.,0.,0.));
#18125=DIRECTION('',(0.,0.,-1.));
#18126=DIRECTION('center_axis',(0.,0.,1.));
#18127=DIRECTION('ref_axis',(1.,0.,0.));
#18128=DIRECTION('',(0.,0.,1.));
#18129=DIRECTION('center_axis',(0.,0.,-1.));
#18130=DIRECTION('ref_axis',(1.,0.,0.));
#18131=DIRECTION('center_axis',(0.,0.,1.));
#18132=DIRECTION('ref_axis',(1.,0.,0.));
#18133=DIRECTION('',(0.,0.,1.));
#18134=DIRECTION('center_axis',(0.,0.,1.));
#18135=DIRECTION('ref_axis',(1.,0.,0.));
#18136=DIRECTION('',(1.,0.,0.));
#18137=DIRECTION('center_axis',(0.,0.,1.));
#18138=DIRECTION('ref_axis',(1.,0.,0.));
#18139=DIRECTION('center_axis',(0.,0.,1.));
#18140=DIRECTION('ref_axis',(1.,0.,0.));
#18141=DIRECTION('',(0.,0.,-1.));
#18142=DIRECTION('center_axis',(0.,0.,1.));
#18143=DIRECTION('ref_axis',(1.,0.,0.));
#18144=DIRECTION('',(0.,0.,1.));
#18145=DIRECTION('center_axis',(0.,0.,-1.));
#18146=DIRECTION('ref_axis',(1.,0.,0.));
#18147=DIRECTION('center_axis',(0.,0.,1.));
#18148=DIRECTION('ref_axis',(1.,0.,0.));
#18149=DIRECTION('',(0.,0.,1.));
#18150=DIRECTION('center_axis',(0.,-1.,0.));
#18151=DIRECTION('ref_axis',(0.,0.,-1.));
#18152=DIRECTION('',(-1.,0.,0.));
#18153=DIRECTION('',(-1.,0.,0.));
#18154=DIRECTION('',(0.,0.,1.));
#18155=DIRECTION('',(1.,0.,0.));
#18156=DIRECTION('',(0.,0.,-1.));
#18157=DIRECTION('',(-1.,0.,0.));
#18158=DIRECTION('center_axis',(0.,1.,0.));
#18159=DIRECTION('ref_axis',(0.,0.,1.));
#18160=DIRECTION('',(1.,0.,0.));
#18161=DIRECTION('',(1.,0.,0.));
#18162=DIRECTION('',(0.,0.,1.));
#18163=DIRECTION('',(1.,0.,0.));
#18164=DIRECTION('',(0.,0.,-1.));
#18165=DIRECTION('',(1.,0.,0.));
#18166=DIRECTION('center_axis',(-1.,0.,0.));
#18167=DIRECTION('ref_axis',(0.,0.,1.));
#18168=DIRECTION('',(0.,-1.,0.));
#18169=DIRECTION('',(0.,0.,1.));
#18170=DIRECTION('',(0.,1.,0.));
#18171=DIRECTION('',(0.,0.,-1.));
#18172=DIRECTION('',(0.,-1.,0.));
#18173=DIRECTION('',(0.,-1.,0.));
#18174=DIRECTION('',(0.,0.,1.));
#18175=DIRECTION('',(0.,-1.,0.));
#18176=DIRECTION('',(0.,0.,-1.));
#18177=DIRECTION('',(0.,-1.,0.));
#18178=DIRECTION('center_axis',(0.,0.,-1.));
#18179=DIRECTION('ref_axis',(0.,1.,0.));
#18180=DIRECTION('',(0.,1.,0.));
#18181=DIRECTION('',(1.,0.,0.));
#18182=DIRECTION('center_axis',(0.,-1.,0.));
#18183=DIRECTION('ref_axis',(0.,0.,-1.));
#18184=DIRECTION('',(0.,0.,-1.));
#18185=DIRECTION('',(1.,0.,0.));
#18186=DIRECTION('center_axis',(0.,0.,1.));
#18187=DIRECTION('ref_axis',(0.,-1.,0.));
#18188=DIRECTION('',(0.,-1.,0.));
#18189=DIRECTION('',(1.,0.,0.));
#18190=DIRECTION('center_axis',(0.,1.,0.));
#18191=DIRECTION('ref_axis',(0.,0.,1.));
#18192=DIRECTION('',(0.,0.,1.));
#18193=DIRECTION('',(1.,0.,0.));
#18194=DIRECTION('center_axis',(0.,0.,-1.));
#18195=DIRECTION('ref_axis',(0.,1.,0.));
#18196=DIRECTION('',(0.,1.,0.));
#18197=DIRECTION('center_axis',(0.,0.,-1.));
#18198=DIRECTION('ref_axis',(0.,1.,0.));
#18199=DIRECTION('',(0.,1.,0.));
#18200=DIRECTION('',(1.,0.,0.));
#18201=DIRECTION('center_axis',(0.,-1.,0.));
#18202=DIRECTION('ref_axis',(0.,0.,-1.));
#18203=DIRECTION('',(0.,0.,-1.));
#18204=DIRECTION('',(1.,0.,0.));
#18205=DIRECTION('center_axis',(0.,0.,-1.));
#18206=DIRECTION('ref_axis',(0.,1.,0.));
#18207=DIRECTION('',(0.,1.,0.));
#18208=DIRECTION('',(1.,0.,0.));
#18209=DIRECTION('center_axis',(0.,1.,0.));
#18210=DIRECTION('ref_axis',(0.,0.,1.));
#18211=DIRECTION('',(0.,0.,1.));
#18212=DIRECTION('',(1.,0.,0.));
#18213=DIRECTION('center_axis',(0.,0.,-1.));
#18214=DIRECTION('ref_axis',(0.,1.,0.));
#18215=DIRECTION('',(0.,1.,0.));
#18216=DIRECTION('center_axis',(1.,0.,0.));
#18217=DIRECTION('ref_axis',(0.,0.,-1.));
#22254=CARTESIAN_POINT('',(0.,0.,0.));
#22255=CARTESIAN_POINT('Origin',(1.5,-1.9,1.7));
#22256=CARTESIAN_POINT('',(1.56403124237433,-1.7,1.7));
#22257=CARTESIAN_POINT('',(1.43596875762567,-1.7,1.7));
#22258=CARTESIAN_POINT('',(0.75,-1.7,1.7));
#22259=CARTESIAN_POINT('Origin',(1.5,-1.9,1.7));
#22260=CARTESIAN_POINT('Origin',(1.5,-1.9,1.7));
#22261=CARTESIAN_POINT('',(1.56403124237433,-1.7,1.75));
#22262=CARTESIAN_POINT('',(1.56403124237433,-1.7,1.7));
#22263=CARTESIAN_POINT('',(1.29,-1.9,1.75));
#22264=CARTESIAN_POINT('Origin',(1.5,-1.9,1.75));
#22265=CARTESIAN_POINT('',(1.29,-1.9,2.4));
#22266=CARTESIAN_POINT('',(1.29,-1.9,1.7));
#22267=CARTESIAN_POINT('Origin',(1.5,-1.9,2.4));
#22268=CARTESIAN_POINT('',(1.43596875762567,-1.7,1.75));
#22269=CARTESIAN_POINT('Origin',(1.5,-1.9,1.75));
#22270=CARTESIAN_POINT('',(1.43596875762567,-1.7,1.7));
#22271=CARTESIAN_POINT('Origin',(-1.5,1.9,1.7));
#22272=CARTESIAN_POINT('',(-1.56403124237433,1.7,1.7));
#22273=CARTESIAN_POINT('',(-1.43596875762567,1.7,1.7));
#22274=CARTESIAN_POINT('',(-0.75,1.7,1.7));
#22275=CARTESIAN_POINT('Origin',(-1.5,1.9,1.7));
#22276=CARTESIAN_POINT('Origin',(-1.5,1.9,1.7));
#22277=CARTESIAN_POINT('',(-1.56403124237433,1.7,1.75));
#22278=CARTESIAN_POINT('',(-1.56403124237433,1.7,1.7));
#22279=CARTESIAN_POINT('',(-1.71,1.9,1.75));
#22280=CARTESIAN_POINT('Origin',(-1.5,1.9,1.75));
#22281=CARTESIAN_POINT('',(-1.71,1.9,2.4));
#22282=CARTESIAN_POINT('',(-1.71,1.9,1.7));
#22283=CARTESIAN_POINT('Origin',(-1.5,1.9,2.4));
#22284=CARTESIAN_POINT('',(-1.43596875762567,1.7,1.75));
#22285=CARTESIAN_POINT('Origin',(-1.5,1.9,1.75));
#22286=CARTESIAN_POINT('',(-1.43596875762567,1.7,1.7));
#22287=CARTESIAN_POINT('Origin',(-1.5,-1.9,1.7));
#22288=CARTESIAN_POINT('',(-1.43596875762567,-1.7,1.7));
#22289=CARTESIAN_POINT('',(-1.56403124237433,-1.7,1.7));
#22290=CARTESIAN_POINT('',(-0.75,-1.7,1.7));
#22291=CARTESIAN_POINT('Origin',(-1.5,-1.9,1.7));
#22292=CARTESIAN_POINT('Origin',(-1.5,-1.9,1.7));
#22293=CARTESIAN_POINT('',(-1.43596875762567,-1.7,1.75));
#22294=CARTESIAN_POINT('',(-1.43596875762567,-1.7,1.7));
#22295=CARTESIAN_POINT('',(-1.71,-1.9,1.75));
#22296=CARTESIAN_POINT('Origin',(-1.5,-1.9,1.75));
#22297=CARTESIAN_POINT('',(-1.71,-1.9,2.4));
#22298=CARTESIAN_POINT('',(-1.71,-1.9,1.7));
#22299=CARTESIAN_POINT('Origin',(-1.5,-1.9,2.4));
#22300=CARTESIAN_POINT('',(-1.56403124237433,-1.7,1.75));
#22301=CARTESIAN_POINT('Origin',(-1.5,-1.9,1.75));
#22302=CARTESIAN_POINT('',(-1.56403124237433,-1.7,1.7));
#22303=CARTESIAN_POINT('Origin',(1.5,1.9,1.7));
#22304=CARTESIAN_POINT('',(1.43596875762567,1.7,1.7));
#22305=CARTESIAN_POINT('',(1.56403124237433,1.7,1.7));
#22306=CARTESIAN_POINT('',(0.75,1.7,1.7));
#22307=CARTESIAN_POINT('Origin',(1.5,1.9,1.7));
#22308=CARTESIAN_POINT('Origin',(1.5,1.9,1.7));
#22309=CARTESIAN_POINT('',(1.43596875762567,1.7,1.75));
#22310=CARTESIAN_POINT('',(1.43596875762567,1.7,1.7));
#22311=CARTESIAN_POINT('',(1.29,1.9,1.75));
#22312=CARTESIAN_POINT('Origin',(1.5,1.9,1.75));
#22313=CARTESIAN_POINT('',(1.29,1.9,2.4));
#22314=CARTESIAN_POINT('',(1.29,1.9,1.7));
#22315=CARTESIAN_POINT('Origin',(1.5,1.9,2.4));
#22316=CARTESIAN_POINT('',(1.56403124237433,1.7,1.75));
#22317=CARTESIAN_POINT('Origin',(1.5,1.9,1.75));
#22318=CARTESIAN_POINT('',(1.56403124237433,1.7,1.7));
#22319=CARTESIAN_POINT('Origin',(0.,-1.7,1.75));
#22320=CARTESIAN_POINT('',(0.,-1.7,1.75));
#22321=CARTESIAN_POINT('',(-1.97,-1.7,1.75));
#22322=CARTESIAN_POINT('',(0.,-1.7,1.75));
#22323=CARTESIAN_POINT('',(-1.97,-1.7,0.43));
#22324=CARTESIAN_POINT('',(-1.97,-1.7,1.75));
#22325=CARTESIAN_POINT('',(1.97,-1.7,0.43));
#22326=CARTESIAN_POINT('',(0.,-1.7,0.43));
#22327=CARTESIAN_POINT('',(1.97,-1.7,1.75));
#22328=CARTESIAN_POINT('',(1.97,-1.7,1.75));
#22329=CARTESIAN_POINT('',(0.,-1.7,1.75));
#22330=CARTESIAN_POINT('Origin',(0.,1.7,0.43));
#22331=CARTESIAN_POINT('',(0.,1.7,1.75));
#22332=CARTESIAN_POINT('',(1.97,1.7,1.75));
#22333=CARTESIAN_POINT('',(0.,1.7,1.75));
#22334=CARTESIAN_POINT('',(1.97,1.7,0.43));
#22335=CARTESIAN_POINT('',(1.97,1.7,0.43));
#22336=CARTESIAN_POINT('',(-1.97,1.7,0.43));
#22337=CARTESIAN_POINT('',(0.,1.7,0.43));
#22338=CARTESIAN_POINT('',(-1.97,1.7,1.75));
#22339=CARTESIAN_POINT('',(-1.97,1.7,0.43));
#22340=CARTESIAN_POINT('',(0.,1.7,1.75));
#22341=CARTESIAN_POINT('Origin',(-1.97,0.,1.415));
#22342=CARTESIAN_POINT('',(-1.97,-2.35,1.75));
#22343=CARTESIAN_POINT('',(-1.97,-2.35,1.75));
#22344=CARTESIAN_POINT('',(-1.97,-2.35,2.4));
#22345=CARTESIAN_POINT('',(-1.97,-2.35,2.4));
#22346=CARTESIAN_POINT('',(-1.97,2.35,2.4));
#22347=CARTESIAN_POINT('',(-1.97,2.35,2.4));
#22348=CARTESIAN_POINT('',(-1.97,2.35,1.75));
#22349=CARTESIAN_POINT('',(-1.97,2.35,1.75));
#22350=CARTESIAN_POINT('',(-1.97,1.7,1.75));
#22351=CARTESIAN_POINT('',(-1.97,0.78,0.43));
#22352=CARTESIAN_POINT('',(-1.97,0.78,0.43));
#22353=CARTESIAN_POINT('',(-1.97,0.78,1.55));
#22354=CARTESIAN_POINT('',(-1.97,0.78,1.55));
#22355=CARTESIAN_POINT('',(-1.97,-0.78,1.55));
#22356=CARTESIAN_POINT('',(-1.97,-0.78,1.55));
#22357=CARTESIAN_POINT('',(-1.97,-0.78,0.43));
#22358=CARTESIAN_POINT('',(-1.97,-0.78,0.43));
#22359=CARTESIAN_POINT('',(-1.97,-1.7,0.43));
#22360=CARTESIAN_POINT('Origin',(0.,-2.35,1.75));
#22361=CARTESIAN_POINT('',(1.97,-2.35,1.75));
#22362=CARTESIAN_POINT('',(1.97,-2.35,1.75));
#22363=CARTESIAN_POINT('',(0.,-2.35,1.75));
#22364=CARTESIAN_POINT('Origin',(0.,-2.35,2.4));
#22365=CARTESIAN_POINT('',(1.97,-2.35,2.4));
#22366=CARTESIAN_POINT('',(1.97,-2.35,2.4));
#22367=CARTESIAN_POINT('',(0.,-2.35,2.4));
#22368=CARTESIAN_POINT('Origin',(0.,2.35,2.4));
#22369=CARTESIAN_POINT('',(1.97,2.35,2.4));
#22370=CARTESIAN_POINT('',(1.97,2.35,2.4));
#22371=CARTESIAN_POINT('',(0.,2.35,2.4));
#22372=CARTESIAN_POINT('Origin',(0.,2.35,1.75));
#22373=CARTESIAN_POINT('',(1.97,2.35,1.75));
#22374=CARTESIAN_POINT('',(1.97,2.35,1.75));
#22375=CARTESIAN_POINT('',(0.,2.35,1.75));
#22376=CARTESIAN_POINT('Origin',(0.,1.7,1.75));
#22377=CARTESIAN_POINT('',(1.97,1.7,1.75));
#22378=CARTESIAN_POINT('Origin',(0.,0.78,0.43));
#22379=CARTESIAN_POINT('',(1.97,0.78,0.43));
#22380=CARTESIAN_POINT('',(1.97,0.78,0.43));
#22381=CARTESIAN_POINT('',(0.,0.78,0.43));
#22382=CARTESIAN_POINT('Origin',(0.,0.78,1.55));
#22383=CARTESIAN_POINT('',(1.97,0.78,1.55));
#22384=CARTESIAN_POINT('',(1.97,0.78,1.55));
#22385=CARTESIAN_POINT('',(0.,0.78,1.55));
#22386=CARTESIAN_POINT('Origin',(0.,-0.78,1.55));
#22387=CARTESIAN_POINT('',(1.97,-0.78,1.55));
#22388=CARTESIAN_POINT('',(1.97,-0.78,1.55));
#22389=CARTESIAN_POINT('',(0.,-0.78,1.55));
#22390=CARTESIAN_POINT('Origin',(0.,-0.78,0.43));
#22391=CARTESIAN_POINT('',(1.97,-0.78,0.43));
#22392=CARTESIAN_POINT('',(1.97,-0.78,0.43));
#22393=CARTESIAN_POINT('',(0.,-0.78,0.43));
#22394=CARTESIAN_POINT('Origin',(0.,-1.7,0.43));
#22395=CARTESIAN_POINT('',(1.97,-1.7,0.43));
#22396=CARTESIAN_POINT('Origin',(1.97,0.,1.415));
#34776=UNCERTAINTY_MEASURE_WITH_UNIT(LENGTH_MEASURE(0.001),#34852,
'DISTANCE_ACCURACY_VALUE',
'Maximum model space distance between geometric entities at asserted c
onnectivities');
#34797=UNCERTAINTY_MEASURE_WITH_UNIT(LENGTH_MEASURE(0.001),#34852,
'DISTANCE_ACCURACY_VALUE',
'Maximum model space distance between geometric entities at asserted c
onnectivities');
#34830=(
GEOMETRIC_REPRESENTATION_CONTEXT(3)
GLOBAL_UNCERTAINTY_ASSIGNED_CONTEXT((#34776))
GLOBAL_UNIT_ASSIGNED_CONTEXT((#34852,#34854,#34855))
REPRESENTATION_CONTEXT('','3D')
);
#34851=(
GEOMETRIC_REPRESENTATION_CONTEXT(3)
GLOBAL_UNCERTAINTY_ASSIGNED_CONTEXT((#34797))
GLOBAL_UNIT_ASSIGNED_CONTEXT((#34852,#34854,#34855))
REPRESENTATION_CONTEXT('','3D')
);
#34852=(
LENGTH_UNIT()
NAMED_UNIT(*)
SI_UNIT(.CENTI.,.METRE.)
);
#34854=(
NAMED_UNIT(*)
PLANE_ANGLE_UNIT()
SI_UNIT($,.RADIAN.)
);
#34855=(
NAMED_UNIT(*)
SI_UNIT($,.STERADIAN.)
SOLID_ANGLE_UNIT()
);
#34888=SHAPE_DEFINITION_REPRESENTATION(#34946,#35105);
#34946=PRODUCT_DEFINITION_SHAPE('',$,#35159);
#35105=SHAPE_REPRESENTATION('',(#15110),#34830);
#35126=PRODUCT_DEFINITION_CONTEXT('part definition',#35287,'design');
#35159=PRODUCT_DEFINITION('Block','Block',#35212,#35126);
#35212=PRODUCT_DEFINITION_FORMATION('',$,#35321);
#35287=APPLICATION_CONTEXT(
'Core Data for Automotive Mechanical Design Process');
#35288=PRODUCT_CONTEXT('part definition',#35287,'mechanical');
#35321=PRODUCT('Block','Block','Block',(#35288));
#35384=COLOUR_RGB('Dark Blue',0.08,0.2,0.34);
#35385=FILL_AREA_STYLE_COLOUR('',#35384);
#35386=FILL_AREA_STYLE('',(#35385));
#35387=SURFACE_STYLE_FILL_AREA(#35386);
#35388=SURFACE_SIDE_STYLE('',(#35387));
#35389=SURFACE_STYLE_USAGE(.BOTH.,#35388);
#35390=PRESENTATION_STYLE_ASSIGNMENT((#35389));
ENDSEC;
END-ISO-10303-21;
